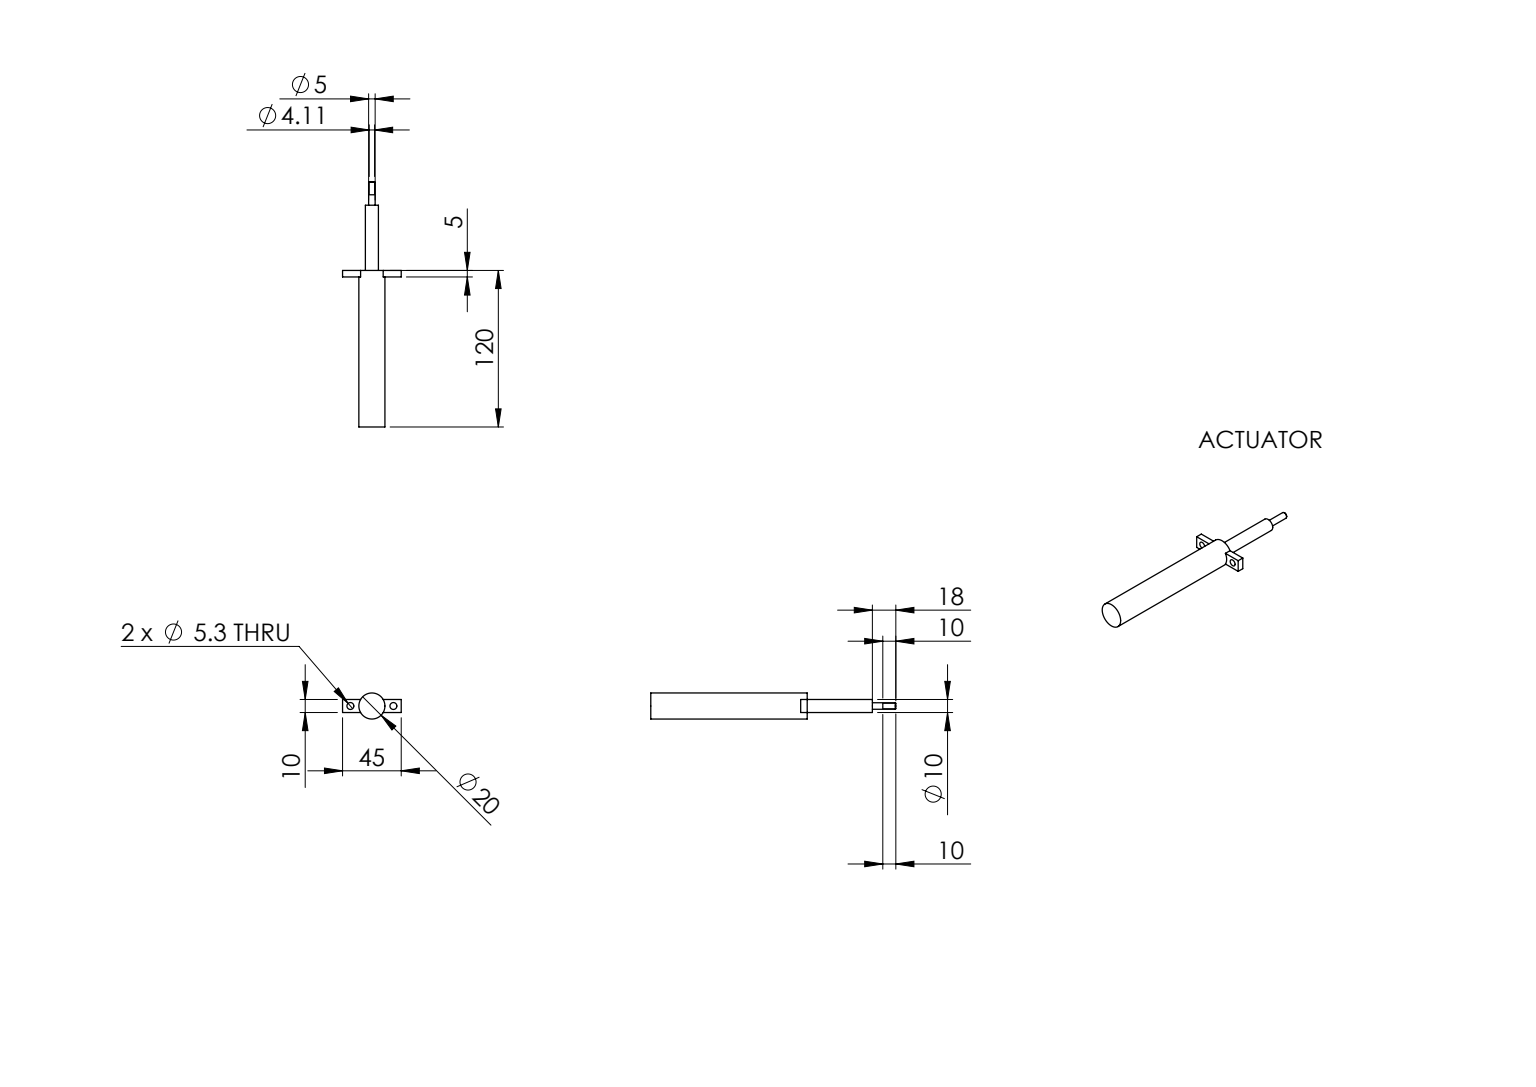
ISO-10303-21;
HEADER;
FILE_DESCRIPTION (('STEP AP214'),
    '1' );
FILE_NAME ('actuator.step',
    '2026-10-24T13:33:06',
    ( '' ),
    ( '' ),
    'SwSTEP 2.0',
    'SolidWorks 2026',
    '' );
FILE_SCHEMA (( 'AUTOMOTIVE_DESIGN' ));
ENDSEC;

DATA;
#20=DIRECTION ( 'NONE',  ( 1.000000000000000000, 0.000000000000000000, 0.000000000000000000 ) ) ;
#34=EDGE_CURVE ( 'NONE', #3584, #3648, #12190, .T. ) ;
#121=ORIENTED_EDGE ( 'NONE', *, *, #4725, .F. ) ;
#127=DIRECTION ( 'NONE',  ( 0.000000000000000000, 0.000000000000000000, 1.000000000000000000 ) ) ;
#157=DIRECTION ( 'NONE',  ( -0.000000000000000000, -0.000000000000000000, 1.000000000000000000 ) ) ;
#162=DIRECTION ( 'NONE',  ( -0.000000000000000000, -0.000000000000000000, 1.000000000000000000 ) ) ;
#163=ADVANCED_FACE ( 'NONE', ( #5247 ), #3288, .T. ) ;
#168=VECTOR ( 'NONE', #12487, 1000.000000000000000 ) ;
#188=EDGE_CURVE ( 'NONE', #1051, #13344, #1074, .T. ) ;
#210=ORIENTED_EDGE ( 'NONE', *, *, #2503, .T. ) ;
#258=VERTEX_POINT ( 'NONE', #13414 ) ;
#274=CARTESIAN_POINT ( 'NONE',  ( 242.5000000000000000, -90.00000000000007105, 55.00000000000001421 ) ) ;
#298=VERTEX_POINT ( 'NONE', #6685 ) ;
#306=EDGE_LOOP ( 'NONE', ( #4499, #12572, #12024, #6931 ) ) ;
#343=ORIENTED_EDGE ( 'NONE', *, *, #8371, .F. ) ;
#394=ADVANCED_FACE ( 'NONE', ( #11247 ), #10594, .F. ) ;
#443=EDGE_CURVE ( 'NONE', #12712, #546, #11238, .T. ) ;
#468=SURFACE_SIDE_STYLE ('',( #3620 ) ) ;
#480=EDGE_LOOP ( 'NONE', ( #9749, #7641, #121, #4547, #3837, #13911, #3499, #11062 ) ) ;
#501=EDGE_LOOP ( 'NONE', ( #3700, #503, #1246, #7982 ) ) ;
#503=ORIENTED_EDGE ( 'NONE', *, *, #10674, .T. ) ;
#509=CIRCLE ( 'NONE', #8650, 9.999999999999980460 ) ;
#531=EDGE_CURVE ( 'NONE', #10688, #3025, #6522, .T. ) ;
#540=CARTESIAN_POINT ( 'NONE',  ( 203.5000000000000000, -85.00000000000007105, 55.00000000000001421 ) ) ;
#546=VERTEX_POINT ( 'NONE', #7599 ) ;
#572=ORIENTED_EDGE ( 'NONE', *, *, #8259, .T. ) ;
#613=EDGE_CURVE ( 'NONE', #4926, #11608, #3124, .T. ) ;
#636=( GEOMETRIC_REPRESENTATION_CONTEXT ( 3 ) GLOBAL_UNCERTAINTY_ASSIGNED_CONTEXT ( ( #7199 ) ) GLOBAL_UNIT_ASSIGNED_CONTEXT ( ( #9242, #8209, #12578 ) ) REPRESENTATION_CONTEXT ( 'NONE', 'WORKASPACE' ) );
#649=VERTEX_POINT ( 'NONE', #8693 ) ;
#674=DIRECTION ( 'NONE',  ( 0.000000000000000000, 0.000000000000000000, -1.000000000000000000 ) ) ;
#682=VERTEX_POINT ( 'NONE', #2166 ) ;
#685=EDGE_CURVE ( 'NONE', #13286, #10688, #9930, .T. ) ;
#743=CARTESIAN_POINT ( 'NONE',  ( 214.9999999999999716, -85.00000000000007105, 64.14213562373096522 ) ) ;
#776=VECTOR ( 'NONE', #9953, 1000.000000000000000 ) ;
#791=VERTEX_POINT ( 'NONE', #4709 ) ;
#799=ADVANCED_FACE ( 'NONE', ( #1417 ), #12246, .F. ) ;
#836=VECTOR ( 'NONE', #2195, 1000.000000000000000 ) ;
#851=ORIENTED_EDGE ( 'NONE', *, *, #1764, .T. ) ;
#856=CARTESIAN_POINT ( 'NONE',  ( 197.5000000000000000, -90.00000000000007105, 55.00000000000001421 ) ) ;
#858=ORIENTED_EDGE ( 'NONE', *, *, #443, .F. ) ;
#859=DIRECTION ( 'NONE',  ( -0.000000000000000000, -0.000000000000000000, -1.000000000000000000 ) ) ;
#867=ORIENTED_EDGE ( 'NONE', *, *, #6061, .T. ) ;
#954=LINE ( 'NONE', #743, #10862 ) ;
#958=CYLINDRICAL_SURFACE ( 'NONE', #7666, 2.649999999999985700 ) ;
#968=EDGE_CURVE ( 'NONE', #546, #10685, #4921, .T. ) ;
#976=ADVANCED_FACE ( 'NONE', ( #12961, #7516, #14185, #4044 ), #6438, .F. ) ;
#978=DIRECTION ( 'NONE',  ( -0.000000000000000000, -0.000000000000000000, 1.000000000000000000 ) ) ;
#996=DIRECTION ( 'NONE',  ( -1.000000000000000000, -2.775557561562893323E-15, 0.000000000000000000 ) ) ;
#1005=DIRECTION ( 'NONE',  ( -0.000000000000000000, -0.000000000000000000, -1.000000000000000000 ) ) ;
#1051=VERTEX_POINT ( 'NONE', #5213 ) ;
#1074=LINE ( 'NONE', #5527, #776 ) ;
#1077=CARTESIAN_POINT ( 'NONE',  ( 229.9999999999999432, -85.00000000000007105, 170.0000000000000000 ) ) ;
#1113=PLANE ( 'NONE',  #4657 ) ;
#1114=FACE_OUTER_BOUND ( 'NONE', #12708, .T. ) ;
#1130=ADVANCED_FACE ( 'NONE', ( #2636, #11413 ), #1113, .F. ) ;
#1180=ORIENTED_EDGE ( 'NONE', *, *, #12121, .F. ) ;
#1212=DIRECTION ( 'NONE',  ( -1.000000000000000000, 0.000000000000000000, 0.000000000000000000 ) ) ;
#1217=DIRECTION ( 'NONE',  ( 2.775557561562893323E-15, -1.000000000000000000, 0.000000000000000000 ) ) ;
#1245=CARTESIAN_POINT ( 'NONE',  ( 233.8499999999999375, -85.00000000000007105, 55.00000000000001421 ) ) ;
#1246=ORIENTED_EDGE ( 'NONE', *, *, #7530, .T. ) ;
#1271=DIRECTION ( 'NONE',  ( 0.000000000000000000, 1.000000000000000000, 0.000000000000000000 ) ) ;
#1280=CARTESIAN_POINT ( 'NONE',  ( 210.0000000000000000, -85.00000000000007105, 55.00000000000002132 ) ) ;
#1282=DIRECTION ( 'NONE',  ( -0.000000000000000000, -0.000000000000000000, 1.000000000000000000 ) ) ;
#1325=CIRCLE ( 'NONE', #11073, 2.649999999999985700 ) ;
#1326=VECTOR ( 'NONE', #5102, 1000.000000000000000 ) ;
#1334=ADVANCED_FACE ( 'NONE', ( #13791, #8424 ), #3863, .F. ) ;
#1403=AXIS2_PLACEMENT_3D ( 'NONE', #4738, #1592, #4667 ) ;
#1410=( GEOMETRIC_REPRESENTATION_CONTEXT ( 3 ) GLOBAL_UNCERTAINTY_ASSIGNED_CONTEXT ( ( #13197 ) ) GLOBAL_UNIT_ASSIGNED_CONTEXT ( ( #9062, #3423, #3835 ) ) REPRESENTATION_CONTEXT ( 'NONE', 'WORKASPACE' ) );
#1411=DIRECTION ( 'NONE',  ( -1.000000000000000000, 0.000000000000000000, 0.000000000000000000 ) ) ;
#1417=FACE_OUTER_BOUND ( 'NONE', #5088, .T. ) ;
#1427=EDGE_CURVE ( 'NONE', #12703, #13122, #7623, .T. ) ;
#1453=DIRECTION ( 'NONE',  ( 1.000000000000000000, 0.000000000000000000, 0.000000000000000000 ) ) ;
#1463=ORIENTED_EDGE ( 'NONE', *, *, #4765, .F. ) ;
#1483=DIRECTION ( 'NONE',  ( 1.000000000000000000, 0.000000000000000000, 0.000000000000000000 ) ) ;
#1486=CARTESIAN_POINT ( 'NONE',  ( 219.9999999999999147, -85.00000000000009948, -17.55500000000000327 ) ) ;
#1489=EDGE_CURVE ( 'NONE', #11495, #5325, #5454, .T. ) ;
#1545=AXIS2_PLACEMENT_3D ( 'NONE', #4006, #10533, #9520 ) ;
#1552=FACE_OUTER_BOUND ( 'NONE', #13347, .T. ) ;
#1562=ORIENTED_EDGE ( 'NONE', *, *, #10674, .F. ) ;
#1580=ORIENTED_EDGE ( 'NONE', *, *, #6064, .T. ) ;
#1592=DIRECTION ( 'NONE',  ( 0.000000000000000000, -1.000000000000000000, 0.000000000000000000 ) ) ;
#1594=CARTESIAN_POINT ( 'NONE',  ( 206.1500000000000057, -85.00000000000007105, 55.00000000000001421 ) ) ;
#1627=FACE_OUTER_BOUND ( 'NONE', #2552, .T. ) ;
#1637=CARTESIAN_POINT ( 'NONE',  ( 222.0549999999999216, -85.00000000000009948, -18.00000000000000355 ) ) ;
#1642=FACE_OUTER_BOUND ( 'NONE', #13415, .T. ) ;
#1654=DIRECTION ( 'NONE',  ( 1.000000000000000000, 0.000000000000000000, 0.000000000000000000 ) ) ;
#1702=ORIENTED_EDGE ( 'NONE', *, *, #4765, .T. ) ;
#1703=CARTESIAN_POINT ( 'NONE',  ( 219.9999999999999716, -85.00000000000007105, 170.0000000000000000 ) ) ;
#1762=AXIS2_PLACEMENT_3D ( 'NONE', #10106, #12144, #3519 ) ;
#1764=EDGE_CURVE ( 'NONE', #649, #298, #8332, .T. ) ;
#1788=EDGE_LOOP ( 'NONE', ( #3445, #8098, #4357, #6788 ) ) ;
#1793=DIRECTION ( 'NONE',  ( 1.000000000000000000, 0.000000000000000000, 0.000000000000000000 ) ) ;
#1802=EDGE_LOOP ( 'NONE', ( #7587, #12705 ) ) ;
#1805=EDGE_LOOP ( 'NONE', ( #3227, #10313 ) ) ;
#1861=AXIS2_PLACEMENT_3D ( 'NONE', #3908, #10435, #11668 ) ;
#1870=PRODUCT_DEFINITION ( 'UNKNOWN', '', #8642, #2767 ) ;
#1881=VERTEX_POINT ( 'NONE', #5371 ) ;
#2003=CIRCLE ( 'NONE', #14082, 2.649999999999985700 ) ;
#2050=CARTESIAN_POINT ( 'NONE',  ( 219.9999999999999147, -85.00000000000009948, -17.55500000000000327 ) ) ;
#2052=CARTESIAN_POINT ( 'NONE',  ( 200.8500000000000227, -85.00000000000007105, 50.00000000000001421 ) ) ;
#2054=EDGE_CURVE ( 'NONE', #13344, #10688, #7295, .T. ) ;
#2062=ORIENTED_EDGE ( 'NONE', *, *, #1427, .F. ) ;
#2152=EDGE_LOOP ( 'NONE', ( #4708, #4758, #4849, #9813, #5810 ) ) ;
#2166=CARTESIAN_POINT ( 'NONE',  ( 228.6602540378443393, -80.00000000000007105, 50.00000000000001421 ) ) ;
#2181=DIRECTION ( 'NONE',  ( -0.000000000000000000, -1.000000000000000000, -0.000000000000000000 ) ) ;
#2183=LINE ( 'NONE', #856, #3860 ) ;
#2195=DIRECTION ( 'NONE',  ( -0.000000000000000000, -0.000000000000000000, 1.000000000000000000 ) ) ;
#2198=DIRECTION ( 'NONE',  ( 0.000000000000000000, 1.000000000000000000, 0.000000000000000000 ) ) ;
#2200=CLOSED_SHELL ( 'NONE', ( #3269, #5695, #3723, #9080, #6131, #163, #11343, #8907, #4814, #1334, #2313, #976, #394, #799, #3827, #1130, #3012, #3741, #6245, #11618, #8182, #11286, #11248, #13792 ) ) ;
#2216=VECTOR ( 'NONE', #10603, 1000.000000000000000 ) ;
#2220=CARTESIAN_POINT ( 'NONE',  ( 228.6602540378443393, -80.00000000000007105, 55.00000000000002132 ) ) ;
#2233=CARTESIAN_POINT ( 'NONE',  ( 197.5000000000000000, -90.00000000000007105, 55.00000000000001421 ) ) ;
#2236=CARTESIAN_POINT ( 'NONE',  ( 219.9999999999999147, -85.00000000000009948, 0.000000000000000000 ) ) ;
#2237=CIRCLE ( 'NONE', #1762, 9.999999999999980460 ) ;
#2250=DIRECTION ( 'NONE',  ( -1.000000000000000000, 0.000000000000000000, 0.000000000000000000 ) ) ;
#2276=VERTEX_POINT ( 'NONE', #5632 ) ;
#2310=EDGE_LOOP ( 'NONE', ( #10390, #4973 ) ) ;
#2313=ADVANCED_FACE ( 'NONE', ( #8604 ), #5418, .T. ) ;
#2343=CARTESIAN_POINT ( 'NONE',  ( 242.5000000000000000, -90.00000000000007105, 55.00000000000001421 ) ) ;
#2374=DIRECTION ( 'NONE',  ( 1.000000000000000000, 0.000000000000000000, 0.000000000000000000 ) ) ;
#2388=CARTESIAN_POINT ( 'NONE',  ( 203.5000000000000000, -85.00000000000007105, 50.00000000000001421 ) ) ;
#2434=DIRECTION ( 'NONE',  ( 1.000000000000000000, 0.000000000000000000, 0.000000000000000000 ) ) ;
#2438=DIRECTION ( 'NONE',  ( -1.000000000000000000, 0.000000000000000000, 0.000000000000000000 ) ) ;
#2442=VECTOR ( 'NONE', #2980, 1000.000000000000000 ) ;
#2448=DIRECTION ( 'NONE',  ( -0.000000000000000000, -0.000000000000000000, 1.000000000000000000 ) ) ;
#2470=AXIS2_PLACEMENT_3D ( 'NONE', #11242, #1282, #9061 ) ;
#2487=VECTOR ( 'NONE', #12138, 1000.000000000000000 ) ;
#2503=EDGE_CURVE ( 'NONE', #3958, #258, #9010, .T. ) ;
#2552=EDGE_LOOP ( 'NONE', ( #4449, #1463, #8826, #1580 ) ) ;
#2566=EDGE_CURVE ( 'NONE', #4150, #298, #9941, .T. ) ;
#2593=DIRECTION ( 'NONE',  ( 1.000000000000000000, 0.000000000000000000, 0.000000000000000000 ) ) ;
#2636=FACE_BOUND ( 'NONE', #1805, .T. ) ;
#2658=EDGE_CURVE ( 'NONE', #3958, #4926, #9300, .T. ) ;
#2668=VECTOR ( 'NONE', #5368, 1000.000000000000000 ) ;
#2690=ORIENTED_EDGE ( 'NONE', *, *, #5877, .T. ) ;
#2693=CARTESIAN_POINT ( 'NONE',  ( 222.0549999999999216, -85.00000000000009948, -18.00000000000000355 ) ) ;
#2714=VECTOR ( 'NONE', #8375, 1000.000000000000000 ) ;
#2741=VERTEX_POINT ( 'NONE', #13500 ) ;
#2767=PRODUCT_DEFINITION_CONTEXT ( 'detailed design', #12304, 'design' ) ;
#2828=CIRCLE ( 'NONE', #10943, 2.500000000000002220 ) ;
#2837=CARTESIAN_POINT ( 'NONE',  ( 242.5000000000000000, -90.00000000000007105, 50.00000000000001421 ) ) ;
#2965=DIRECTION ( 'NONE',  ( 1.000000000000000000, 0.000000000000000000, -0.000000000000000000 ) ) ;
#2980=DIRECTION ( 'NONE',  ( -1.000000000000000000, -0.000000000000000000, -0.000000000000000000 ) ) ;
#3012=ADVANCED_FACE ( 'NONE', ( #4434 ), #8851, .F. ) ;
#3025=VERTEX_POINT ( 'NONE', #14140 ) ;
#3029=DIRECTION ( 'NONE',  ( -1.000000000000000000, 0.000000000000000000, 0.000000000000000000 ) ) ;
#3044=AXIS2_PLACEMENT_3D ( 'NONE', #8830, #12373, #20 ) ;
#3048=CIRCLE ( 'NONE', #13450, 2.055000000000001492 ) ;
#3099=CARTESIAN_POINT ( 'NONE',  ( 219.9999999999999716, -85.00000000000007105, 50.00000000000001421 ) ) ;
#3124=LINE ( 'NONE', #10954, #7740 ) ;
#3168=LINE ( 'NONE', #7360, #2714 ) ;
#3217=VERTEX_POINT ( 'NONE', #1280 ) ;
#3223=ORIENTED_EDGE ( 'NONE', *, *, #11905, .F. ) ;
#3227=ORIENTED_EDGE ( 'NONE', *, *, #8947, .F. ) ;
#3230=FACE_OUTER_BOUND ( 'NONE', #11862, .T. ) ;
#3235=EDGE_CURVE ( 'NONE', #10685, #7175, #9516, .T. ) ;
#3269=ADVANCED_FACE ( 'NONE', ( #1642 ), #11741, .T. ) ;
#3277=DIRECTION ( 'NONE',  ( 0.000000000000000000, 0.000000000000000000, -1.000000000000000000 ) ) ;
#3282=LINE ( 'NONE', #10019, #6027 ) ;
#3288=CYLINDRICAL_SURFACE ( 'NONE', #13312, 9.999999999999980460 ) ;
#3304=FACE_OUTER_BOUND ( 'NONE', #501, .T. ) ;
#3326=VECTOR ( 'NONE', #6308, 1000.000000000000000 ) ;
#3331=CIRCLE ( 'NONE', #8165, 5.000000000000004441 ) ;
#3353=DIRECTION ( 'NONE',  ( 1.000000000000000000, 0.000000000000000000, 0.000000000000000000 ) ) ;
#3362=EDGE_LOOP ( 'NONE', ( #3792, #12684, #11851, #10750 ) ) ;
#3363=DIRECTION ( 'NONE',  ( -1.000000000000000000, 0.000000000000000000, 0.000000000000000000 ) ) ;
#3375=EDGE_LOOP ( 'NONE', ( #9305, #6235 ) ) ;
#3385=SHAPE_REPRESENTATION ( 'actuator', ( #14039 ), #1410 ) ;
#3411=DIRECTION ( 'NONE',  ( 1.000000000000000000, 0.000000000000000000, 0.000000000000000000 ) ) ;
#3423=( NAMED_UNIT ( * ) PLANE_ANGLE_UNIT ( ) SI_UNIT ( $, .RADIAN. ) );
#3439=DIRECTION ( 'NONE',  ( -0.000000000000000000, -0.000000000000000000, 1.000000000000000000 ) ) ;
#3440=DIRECTION ( 'NONE',  ( 1.000000000000000000, 0.000000000000000000, 0.000000000000000000 ) ) ;
#3445=ORIENTED_EDGE ( 'NONE', *, *, #1764, .F. ) ;
#3458=CARTESIAN_POINT ( 'NONE',  ( 242.4999999999999716, -80.00000000000007105, 55.00000000000001421 ) ) ;
#3462=CYLINDRICAL_SURFACE ( 'NONE', #12998, 2.649999999999985700 ) ;
#3466=EDGE_LOOP ( 'NONE', ( #2062, #7298, #14098, #9821, #343, #13771, #1562, #1180 ) ) ;
#3499=ORIENTED_EDGE ( 'NONE', *, *, #4750, .F. ) ;
#3519=DIRECTION ( 'NONE',  ( -1.000000000000000000, 0.000000000000000000, 0.000000000000000000 ) ) ;
#3536=DIRECTION ( 'NONE',  ( -0.000000000000000000, -0.000000000000000000, -1.000000000000000000 ) ) ;
#3561=ORIENTED_EDGE ( 'NONE', *, *, #8052, .T. ) ;
#3584=VERTEX_POINT ( 'NONE', #7278 ) ;
#3602=CYLINDRICAL_SURFACE ( 'NONE', #12776, 2.649999999999985700 ) ;
#3620=SURFACE_STYLE_FILL_AREA ( #12395 ) ;
#3632=ORIENTED_EDGE ( 'NONE', *, *, #11546, .F. ) ;
#3643=CARTESIAN_POINT ( 'NONE',  ( 219.9999999999999716, -85.00000000000007105, 0.000000000000000000 ) ) ;
#3648=VERTEX_POINT ( 'NONE', #2052 ) ;
#3658=EDGE_CURVE ( 'NONE', #649, #13881, #3048, .T. ) ;
#3680=AXIS2_PLACEMENT_3D ( 'NONE', #2050, #8941, #3440 ) ;
#3700=ORIENTED_EDGE ( 'NONE', *, *, #12163, .F. ) ;
#3703=AXIS2_PLACEMENT_3D ( 'NONE', #10869, #10726, #2965 ) ;
#3705=CARTESIAN_POINT ( 'NONE',  ( 239.1499999999999204, -85.00000000000007105, 50.00000000000001421 ) ) ;
#3723=ADVANCED_FACE ( 'NONE', ( #12205 ), #958, .F. ) ;
#3741=ADVANCED_FACE ( 'NONE', ( #3304 ), #10989, .F. ) ;
#3745=CARTESIAN_POINT ( 'NONE',  ( 236.4999999999999432, -85.00000000000007105, 55.00000000000001421 ) ) ;
#3775=DIRECTION ( 'NONE',  ( 1.000000000000000000, 0.000000000000000000, 0.000000000000000000 ) ) ;
#3780=EDGE_LOOP ( 'NONE', ( #12090, #6328, #7485, #8984 ) ) ;
#3787=EDGE_CURVE ( 'NONE', #5325, #2741, #4445, .T. ) ;
#3792=ORIENTED_EDGE ( 'NONE', *, *, #8052, .F. ) ;
#3827=ADVANCED_FACE ( 'NONE', ( #8055 ), #5960, .F. ) ;
#3835=( NAMED_UNIT ( * ) SI_UNIT ( $, .STERADIAN. ) SOLID_ANGLE_UNIT ( ) );
#3837=ORIENTED_EDGE ( 'NONE', *, *, #8504, .T. ) ;
#3860=VECTOR ( 'NONE', #13064, 1000.000000000000000 ) ;
#3863=PLANE ( 'NONE',  #13468 ) ;
#3888=AXIS2_PLACEMENT_3D ( 'NONE', #6533, #14211, #7819 ) ;
#3908=CARTESIAN_POINT ( 'NONE',  ( 236.4999999999999432, -85.00000000000007105, 55.00000000000001421 ) ) ;
#3958=VERTEX_POINT ( 'NONE', #12185 ) ;
#3964=EDGE_CURVE ( 'NONE', #13344, #5408, #3282, .T. ) ;
#3972=PLANE ( 'NONE',  #9753 ) ;
#4006=CARTESIAN_POINT ( 'NONE',  ( 219.9999999999999147, -85.00000000000009948, -17.55500000000000327 ) ) ;
#4035=DIRECTION ( 'NONE',  ( -0.000000000000000000, -0.000000000000000000, -1.000000000000000000 ) ) ;
#4044=FACE_OUTER_BOUND ( 'NONE', #12958, .T. ) ;
#4052=LINE ( 'NONE', #8401, #4402 ) ;
#4083=ORIENTED_EDGE ( 'NONE', *, *, #6289, .T. ) ;
#4099=LINE ( 'NONE', #6128, #11881 ) ;
#4110=CARTESIAN_POINT ( 'NONE',  ( 219.9999999999999716, -85.00000000000007105, 50.00000000000001421 ) ) ;
#4150=VERTEX_POINT ( 'NONE', #8109 ) ;
#4164=DIRECTION ( 'NONE',  ( 1.000000000000000000, 0.000000000000000000, 0.000000000000000000 ) ) ;
#4165=AXIS2_PLACEMENT_3D ( 'NONE', #9623, #674, #14036 ) ;
#4166=DIRECTION ( 'NONE',  ( -0.000000000000000000, -0.000000000000000000, 1.000000000000000000 ) ) ;
#4244=CARTESIAN_POINT ( 'NONE',  ( 210.0000000000000000, -85.00000000000007105, 170.0000000000000000 ) ) ;
#4261=DIRECTION ( 'NONE',  ( 1.000000000000000000, 0.000000000000000000, -0.000000000000000000 ) ) ;
#4287=EDGE_LOOP ( 'NONE', ( #11625, #4346, #13827, #9504 ) ) ;
#4289=DIRECTION ( 'NONE',  ( 0.000000000000000000, -0.000000000000000000, -1.000000000000000000 ) ) ;
#4298=ORIENTED_EDGE ( 'NONE', *, *, #3235, .T. ) ;
#4346=ORIENTED_EDGE ( 'NONE', *, *, #7170, .T. ) ;
#4348=DIRECTION ( 'NONE',  ( -1.000000000000000000, -0.000000000000000000, -0.000000000000000000 ) ) ;
#4357=ORIENTED_EDGE ( 'NONE', *, *, #10565, .T. ) ;
#4386=DIRECTION ( 'NONE',  ( 1.000000000000000000, 0.000000000000000000, 0.000000000000000000 ) ) ;
#4389=CARTESIAN_POINT ( 'NONE',  ( 197.5000000000000000, -90.00000000000007105, 55.00000000000001421 ) ) ;
#4402=VECTOR ( 'NONE', #978, 1000.000000000000000 ) ;
#4434=FACE_OUTER_BOUND ( 'NONE', #3780, .T. ) ;
#4441=ORIENTED_EDGE ( 'NONE', *, *, #11212, .F. ) ;
#4445=CIRCLE ( 'NONE', #8096, 5.000000000000004441 ) ;
#4446=DIRECTION ( 'NONE',  ( -0.000000000000000000, -0.000000000000000000, -1.000000000000000000 ) ) ;
#4449=ORIENTED_EDGE ( 'NONE', *, *, #1489, .F. ) ;
#4469=EDGE_CURVE ( 'NONE', #298, #9222, #4052, .T. ) ;
#4472=ORIENTED_EDGE ( 'NONE', *, *, #11702, .F. ) ;
#4483=DIRECTION ( 'NONE',  ( -1.000000000000000000, 0.000000000000000000, -0.000000000000000000 ) ) ;
#4484=VECTOR ( 'NONE', #10993, 1000.000000000000000 ) ;
#4495=PRODUCT ( 'actuator', 'actuator', '', ( #4956 ) ) ;
#4499=ORIENTED_EDGE ( 'NONE', *, *, #10635, .F. ) ;
#4547=ORIENTED_EDGE ( 'NONE', *, *, #13997, .F. ) ;
#4591=DIRECTION ( 'NONE',  ( -0.000000000000000000, -0.000000000000000000, 1.000000000000000000 ) ) ;
#4595=DIRECTION ( 'NONE',  ( 0.000000000000000000, -0.000000000000000000, 1.000000000000000000 ) ) ;
#4622=CARTESIAN_POINT ( 'NONE',  ( 236.4999999999999432, -85.00000000000007105, 55.00000000000001421 ) ) ;
#4635=ORIENTED_EDGE ( 'NONE', *, *, #6061, .F. ) ;
#4657=AXIS2_PLACEMENT_3D ( 'NONE', #7054, #11084, #4483 ) ;
#4667=DIRECTION ( 'NONE',  ( 0.000000000000000000, -0.000000000000000000, -1.000000000000000000 ) ) ;
#4708=ORIENTED_EDGE ( 'NONE', *, *, #613, .T. ) ;
#4709=CARTESIAN_POINT ( 'NONE',  ( 210.0000000000000000, -85.00000000000007105, 170.0000000000000000 ) ) ;
#4725=EDGE_CURVE ( 'NONE', #11608, #13122, #6473, .T. ) ;
#4738=CARTESIAN_POINT ( 'NONE',  ( 197.5000000000000000, -80.00000000000007105, 55.00000000000001421 ) ) ;
#4750=EDGE_CURVE ( 'NONE', #3217, #1051, #8158, .T. ) ;
#4758=ORIENTED_EDGE ( 'NONE', *, *, #4725, .T. ) ;
#4759=AXIS2_PLACEMENT_3D ( 'NONE', #5349, #7789, #4261 ) ;
#4765=EDGE_CURVE ( 'NONE', #1881, #11495, #7399, .T. ) ;
#4774=DIRECTION ( 'NONE',  ( -0.000000000000000000, -0.000000000000000000, 1.000000000000000000 ) ) ;
#4785=AXIS2_PLACEMENT_3D ( 'NONE', #7078, #10346, #1483 ) ;
#4792=VECTOR ( 'NONE', #8065, 1000.000000000000000 ) ;
#4814=ADVANCED_FACE ( 'NONE', ( #1627 ), #5066, .T. ) ;
#4825=CARTESIAN_POINT ( 'NONE',  ( 200.8500000000000227, -85.00000000000007105, 55.00000000000001421 ) ) ;
#4848=DIRECTION ( 'NONE',  ( -0.000000000000000000, -0.000000000000000000, 1.000000000000000000 ) ) ;
#4849=ORIENTED_EDGE ( 'NONE', *, *, #12121, .T. ) ;
#4853=DIRECTION ( 'NONE',  ( 0.000000000000000000, 0.000000000000000000, -1.000000000000000000 ) ) ;
#4886=ORIENTED_EDGE ( 'NONE', *, *, #2054, .T. ) ;
#4897=LINE ( 'NONE', #9318, #9440 ) ;
#4916=COLOUR_RGB ( '',0.8941176470588234615, 0.8941176470588234615, 0.8941176470588234615 ) ;
#4921=LINE ( 'NONE', #13896, #5342 ) ;
#4926=VERTEX_POINT ( 'NONE', #3458 ) ;
#4956=PRODUCT_CONTEXT ( 'NONE', #6096, 'mechanical' ) ;
#4973=ORIENTED_EDGE ( 'NONE', *, *, #11212, .T. ) ;
#4986=CARTESIAN_POINT ( 'NONE',  ( 219.9999999999999716, -85.00000000000007105, 64.14213562373096522 ) ) ;
#4993=DIRECTION ( 'NONE',  ( -0.000000000000000000, -0.000000000000000000, 1.000000000000000000 ) ) ;
#5013=ORIENTED_EDGE ( 'NONE', *, *, #8715, .F. ) ;
#5019=CIRCLE ( 'NONE', #2470, 2.500000000000002220 ) ;
#5035=AXIS2_PLACEMENT_3D ( 'NONE', #1703, #13676, #11577 ) ;
#5066=CYLINDRICAL_SURFACE ( 'NONE', #8313, 5.000000000000004441 ) ;
#5072=VECTOR ( 'NONE', #11856, 1000.000000000000000 ) ;
#5077=DIRECTION ( 'NONE',  ( 1.000000000000000000, 0.000000000000000000, 0.000000000000000000 ) ) ;
#5088=EDGE_LOOP ( 'NONE', ( #7598, #6594, #6457, #2690 ) ) ;
#5101=EDGE_LOOP ( 'NONE', ( #13141, #5013 ) ) ;
#5102=DIRECTION ( 'NONE',  ( 0.000000000000000000, 0.000000000000000000, 1.000000000000000000 ) ) ;
#5206=ORIENTED_EDGE ( 'NONE', *, *, #34, .T. ) ;
#5213=CARTESIAN_POINT ( 'NONE',  ( 211.3397459621556038, -80.00000000000007105, 55.00000000000002132 ) ) ;
#5245=AXIS2_PLACEMENT_3D ( 'NONE', #2233, #1271, #9118 ) ;
#5247=FACE_OUTER_BOUND ( 'NONE', #480, .T. ) ;
#5258=ADVANCED_BREP_SHAPE_REPRESENTATION ( '', ( #13412, #14039 ), #1410 ) ;
#5264=VECTOR ( 'NONE', #6604, 1000.000000000000000 ) ;
#5309=CARTESIAN_POINT ( 'NONE',  ( 239.1499999999999204, -85.00000000000007105, 55.00000000000001421 ) ) ;
#5325=VERTEX_POINT ( 'NONE', #6124 ) ;
#5342=VECTOR ( 'NONE', #4993, 1000.000000000000000 ) ;
#5349=CARTESIAN_POINT ( 'NONE',  ( 219.9999999999999716, -85.00000000000007105, 170.0000000000000000 ) ) ;
#5368=DIRECTION ( 'NONE',  ( -0.000000000000000000, -1.000000000000000000, -0.000000000000000000 ) ) ;
#5371=CARTESIAN_POINT ( 'NONE',  ( 214.9999999999999716, -85.00000000000007105, 50.00000000000001421 ) ) ;
#5408=VERTEX_POINT ( 'NONE', #4389 ) ;
#5418=PLANE ( 'NONE',  #4759 ) ;
#5454=LINE ( 'NONE', #5599, #10948 ) ;
#5464=LINE ( 'NONE', #4244, #2487 ) ;
#5467=EDGE_CURVE ( 'NONE', #791, #3217, #5464, .T. ) ;
#5468=CARTESIAN_POINT ( 'NONE',  ( 197.5000000000000000, -80.00000000000007105, 50.00000000000001421 ) ) ;
#5512=EDGE_CURVE ( 'NONE', #5681, #13411, #1325, .T. ) ;
#5527=CARTESIAN_POINT ( 'NONE',  ( 197.5000000000000000, -80.00000000000007105, 55.00000000000001421 ) ) ;
#5537=CARTESIAN_POINT ( 'NONE',  ( 219.9999999999999147, -85.00000000000009948, 0.000000000000000000 ) ) ;
#5538=LINE ( 'NONE', #14159, #836 ) ;
#5599=CARTESIAN_POINT ( 'NONE',  ( 224.9999999999999716, -85.00000000000007105, 64.14213562373096522 ) ) ;
#5632=CARTESIAN_POINT ( 'NONE',  ( 211.3397459621556038, -90.00000000000007105, 55.00000000000002132 ) ) ;
#5664=ORIENTED_EDGE ( 'NONE', *, *, #2566, .F. ) ;
#5669=CARTESIAN_POINT ( 'NONE',  ( 203.5000000000000000, -85.00000000000007105, 50.00000000000001421 ) ) ;
#5674=DIRECTION ( 'NONE',  ( -0.000000000000000000, -0.000000000000000000, 1.000000000000000000 ) ) ;
#5681=VERTEX_POINT ( 'NONE', #1594 ) ;
#5695=ADVANCED_FACE ( 'NONE', ( #11690 ), #13137, .T. ) ;
#5701=CARTESIAN_POINT ( 'NONE',  ( 219.9999999999999716, -85.00000000000007105, 170.0000000000000000 ) ) ;
#5722=CARTESIAN_POINT ( 'NONE',  ( 197.5000000000000000, -90.00000000000007105, 55.00000000000001421 ) ) ;
#5737=VERTEX_POINT ( 'NONE', #5964 ) ;
#5748=MECHANICAL_DESIGN_GEOMETRIC_PRESENTATION_REPRESENTATION('',(#10149),#636);
#5796=SHAPE_REPRESENTATION_RELATIONSHIP ( 'NONE' , 'NONE' ,  #3385, #5258 ) ;
#5810=ORIENTED_EDGE ( 'NONE', *, *, #2658, .T. ) ;
#5812=CARTESIAN_POINT ( 'NONE',  ( 222.4999999999999147, -85.00000000000009948, 0.000000000000000000 ) ) ;
#5831=( GEOMETRIC_REPRESENTATION_CONTEXT ( 3 ) GLOBAL_UNCERTAINTY_ASSIGNED_CONTEXT ( ( #7678 ) ) GLOBAL_UNIT_ASSIGNED_CONTEXT ( ( #10513, #11386, #6954 ) ) REPRESENTATION_CONTEXT ( 'NONE', 'WORKASPACE' ) );
#5877=EDGE_CURVE ( 'NONE', #5408, #3025, #2183, .T. ) ;
#5924=DIRECTION ( 'NONE',  ( 0.000000000000000000, 0.000000000000000000, -1.000000000000000000 ) ) ;
#5929=DIRECTION ( 'NONE',  ( 1.000000000000000000, 0.000000000000000000, 0.000000000000000000 ) ) ;
#5960=PLANE ( 'NONE',  #1403 ) ;
#5964=CARTESIAN_POINT ( 'NONE',  ( 211.3397459621556038, -90.00000000000007105, 50.00000000000001421 ) ) ;
#5966=ORIENTED_EDGE ( 'NONE', *, *, #531, .F. ) ;
#5969=AXIS2_PLACEMENT_3D ( 'NONE', #11239, #11107, #3353 ) ;
#5986=EDGE_LOOP ( 'NONE', ( #12619, #12076, #11050, #210 ) ) ;
#6001=FACE_OUTER_BOUND ( 'NONE', #9836, .T. ) ;
#6027=VECTOR ( 'NONE', #2181, 1000.000000000000000 ) ;
#6033=SHAPE_DEFINITION_REPRESENTATION ( #12484, #3385 ) ;
#6036=CONICAL_SURFACE ( 'NONE', #11591, 2.500000000000002220, 0.7853981633974521648 ) ;
#6046=EDGE_LOOP ( 'NONE', ( #5206, #572 ) ) ;
#6059=DIRECTION ( 'NONE',  ( 1.000000000000000000, 0.000000000000000000, 0.000000000000000000 ) ) ;
#6061=EDGE_CURVE ( 'NONE', #13881, #649, #7325, .T. ) ;
#6064=EDGE_CURVE ( 'NONE', #2741, #5325, #8483, .T. ) ;
#6096=APPLICATION_CONTEXT ( 'automotive_design' ) ;
#6124=CARTESIAN_POINT ( 'NONE',  ( 224.9999999999999716, -85.00000000000007105, 0.000000000000000000 ) ) ;
#6128=CARTESIAN_POINT ( 'NONE',  ( 222.4999999999999147, -85.00000000000009948, -17.55500000000000327 ) ) ;
#6131=ADVANCED_FACE ( 'NONE', ( #9480 ), #7228, .T. ) ;
#6132=DIRECTION ( 'NONE',  ( 0.000000000000000000, 0.000000000000000000, 1.000000000000000000 ) ) ;
#6147=PLANE ( 'NONE',  #9041 ) ;
#6182=DIRECTION ( 'NONE',  ( 1.000000000000000000, 0.000000000000000000, -0.000000000000000000 ) ) ;
#6199=EDGE_CURVE ( 'NONE', #5408, #2276, #13407, .T. ) ;
#6235=ORIENTED_EDGE ( 'NONE', *, *, #3787, .F. ) ;
#6241=DIRECTION ( 'NONE',  ( -0.000000000000000000, -0.000000000000000000, -1.000000000000000000 ) ) ;
#6245=ADVANCED_FACE ( 'NONE', ( #8853 ), #10971, .F. ) ;
#6289=EDGE_CURVE ( 'NONE', #298, #4150, #5019, .T. ) ;
#6291=DIRECTION ( 'NONE',  ( 0.000000000000000000, 0.000000000000000000, 1.000000000000000000 ) ) ;
#6308=DIRECTION ( 'NONE',  ( -0.7071067811865502373, 8.659560562354966138E-17, 0.7071067811865447972 ) ) ;
#6328=ORIENTED_EDGE ( 'NONE', *, *, #13997, .T. ) ;
#6329=ORIENTED_EDGE ( 'NONE', *, *, #3964, .F. ) ;
#6361=ORIENTED_EDGE ( 'NONE', *, *, #3964, .T. ) ;
#6365=CARTESIAN_POINT ( 'NONE',  ( 224.9999999999999716, -85.00000000000007105, 50.00000000000001421 ) ) ;
#6407=VECTOR ( 'NONE', #5929, 1000.000000000000000 ) ;
#6431=VECTOR ( 'NONE', #8478, 1000.000000000000000 ) ;
#6438=PLANE ( 'NONE',  #3703 ) ;
#6457=ORIENTED_EDGE ( 'NONE', *, *, #6199, .F. ) ;
#6464=CARTESIAN_POINT ( 'NONE',  ( 197.5000000000000000, -80.00000000000007105, 55.00000000000001421 ) ) ;
#6473=CIRCLE ( 'NONE', #11804, 9.999999999999980460 ) ;
#6500=CARTESIAN_POINT ( 'NONE',  ( 217.4999999999999147, -85.00000000000009948, 0.000000000000000000 ) ) ;
#6501=AXIS2_PLACEMENT_3D ( 'NONE', #8322, #9493, #1793 ) ;
#6522=LINE ( 'NONE', #8623, #2668 ) ;
#6533=CARTESIAN_POINT ( 'NONE',  ( 219.9999999999999716, -85.00000000000007105, 50.00000000000001421 ) ) ;
#6548=CIRCLE ( 'NONE', #8144, 2.649999999999985700 ) ;
#6594=ORIENTED_EDGE ( 'NONE', *, *, #8371, .T. ) ;
#6604=DIRECTION ( 'NONE',  ( 1.000000000000000000, 0.000000000000000000, 0.000000000000000000 ) ) ;
#6649=CARTESIAN_POINT ( 'NONE',  ( 236.4999999999999432, -85.00000000000007105, 55.00000000000001421 ) ) ;
#6685=CARTESIAN_POINT ( 'NONE',  ( 217.4999999999999147, -85.00000000000009948, -17.55500000000000327 ) ) ;
#6704=ORIENTED_EDGE ( 'NONE', *, *, #8018, .F. ) ;
#6738=ORIENTED_EDGE ( 'NONE', *, *, #7024, .T. ) ;
#6776=CARTESIAN_POINT ( 'NONE',  ( 228.6602540378443393, -90.00000000000007105, 170.0000000000000000 ) ) ;
#6788=ORIENTED_EDGE ( 'NONE', *, *, #6289, .F. ) ;
#6823=VERTEX_POINT ( 'NONE', #13221 ) ;
#6835=ORIENTED_EDGE ( 'NONE', *, *, #2566, .T. ) ;
#6931=ORIENTED_EDGE ( 'NONE', *, *, #13208, .F. ) ;
#6933=CARTESIAN_POINT ( 'NONE',  ( 219.9999999999999716, -85.00000000000007105, 55.00000000000002132 ) ) ;
#6947=LINE ( 'NONE', #12538, #6407 ) ;
#6954=( NAMED_UNIT ( * ) SI_UNIT ( $, .STERADIAN. ) SOLID_ANGLE_UNIT ( ) );
#6986=ORIENTED_EDGE ( 'NONE', *, *, #8605, .F. ) ;
#6988=STYLED_ITEM ( 'NONE', ( #9280 ), #5258 ) ;
#7024=EDGE_CURVE ( 'NONE', #4150, #8111, #12409, .T. ) ;
#7050=ORIENTED_EDGE ( 'NONE', *, *, #10635, .T. ) ;
#7054=CARTESIAN_POINT ( 'NONE',  ( 0.000000000000000000, 0.000000000000000000, 55.00000000000001421 ) ) ;
#7070=DIRECTION ( 'NONE',  ( 1.000000000000000000, 0.000000000000000000, 0.000000000000000000 ) ) ;
#7078=CARTESIAN_POINT ( 'NONE',  ( 219.9999999999999716, -85.00000000000007105, 0.000000000000000000 ) ) ;
#7131=ORIENTED_EDGE ( 'NONE', *, *, #9072, .T. ) ;
#7170=EDGE_CURVE ( 'NONE', #1051, #13286, #12556, .T. ) ;
#7175=VERTEX_POINT ( 'NONE', #5309 ) ;
#7199=UNCERTAINTY_MEASURE_WITH_UNIT (LENGTH_MEASURE( 1.000000000000000082E-05 ), #9242, 'distance_accuracy_value', 'NONE');
#7228=CYLINDRICAL_SURFACE ( 'NONE', #8953, 5.000000000000004441 ) ;
#7278=CARTESIAN_POINT ( 'NONE',  ( 206.1500000000000057, -85.00000000000007105, 50.00000000000001421 ) ) ;
#7295=LINE ( 'NONE', #7369, #13660 ) ;
#7298=ORIENTED_EDGE ( 'NONE', *, *, #9072, .F. ) ;
#7325=CIRCLE ( 'NONE', #11974, 2.055000000000001492 ) ;
#7360=CARTESIAN_POINT ( 'NONE',  ( 239.1499999999999204, -85.00000000000007105, 55.00000000000001421 ) ) ;
#7369=CARTESIAN_POINT ( 'NONE',  ( 197.5000000000000000, -80.00000000000007105, 55.00000000000001421 ) ) ;
#7399=CIRCLE ( 'NONE', #11572, 5.000000000000004441 ) ;
#7434=VECTOR ( 'NONE', #6059, 1000.000000000000000 ) ;
#7436=CARTESIAN_POINT ( 'NONE',  ( 197.5000000000000000, -80.00000000000007105, 50.00000000000001421 ) ) ;
#7443=DIRECTION ( 'NONE',  ( -0.000000000000000000, -0.000000000000000000, -1.000000000000000000 ) ) ;
#7477=ORIENTED_EDGE ( 'NONE', *, *, #968, .T. ) ;
#7485=ORIENTED_EDGE ( 'NONE', *, *, #613, .F. ) ;
#7486=CARTESIAN_POINT ( 'NONE',  ( 219.9999999999999716, -85.00000000000007105, 170.0000000000000000 ) ) ;
#7516=FACE_BOUND ( 'NONE', #1802, .T. ) ;
#7530=EDGE_CURVE ( 'NONE', #10602, #258, #6947, .T. ) ;
#7533=ORIENTED_EDGE ( 'NONE', *, *, #4469, .T. ) ;
#7560=VECTOR ( 'NONE', #9471, 1000.000000000000000 ) ;
#7563=DIRECTION ( 'NONE',  ( 1.000000000000000000, 0.000000000000000000, 0.000000000000000000 ) ) ;
#7567=AXIS2_PLACEMENT_3D ( 'NONE', #4622, #162, #2374 ) ;
#7580=AXIS2_PLACEMENT_3D ( 'NONE', #11404, #4591, #11333 ) ;
#7585=AXIS2_PLACEMENT_3D ( 'NONE', #5537, #3439, #12277 ) ;
#7587=ORIENTED_EDGE ( 'NONE', *, *, #443, .T. ) ;
#7598=ORIENTED_EDGE ( 'NONE', *, *, #11702, .T. ) ;
#7599=CARTESIAN_POINT ( 'NONE',  ( 233.8499999999999375, -85.00000000000007105, 50.00000000000001421 ) ) ;
#7623=LINE ( 'NONE', #1077, #11877 ) ;
#7641=ORIENTED_EDGE ( 'NONE', *, *, #1427, .T. ) ;
#7666=AXIS2_PLACEMENT_3D ( 'NONE', #13227, #5674, #4386 ) ;
#7678=UNCERTAINTY_MEASURE_WITH_UNIT (LENGTH_MEASURE( 1.000000000000000082E-05 ), #10513, 'distance_accuracy_value', 'NONE');
#7681=DIRECTION ( 'NONE',  ( 0.000000000000000000, -1.000000000000000000, 0.000000000000000000 ) ) ;
#7701=CARTESIAN_POINT ( 'NONE',  ( 197.5000000000000000, -80.00000000000007105, 50.00000000000001421 ) ) ;
#7740=VECTOR ( 'NONE', #4348, 1000.000000000000000 ) ;
#7789=DIRECTION ( 'NONE',  ( 0.000000000000000000, 0.000000000000000000, 1.000000000000000000 ) ) ;
#7818=CARTESIAN_POINT ( 'NONE',  ( 219.9999999999999716, -85.00000000000007105, 55.00000000000002132 ) ) ;
#7819=DIRECTION ( 'NONE',  ( 1.000000000000000000, 0.000000000000000000, 0.000000000000000000 ) ) ;
#7950=ORIENTED_EDGE ( 'NONE', *, *, #968, .F. ) ;
#7982=ORIENTED_EDGE ( 'NONE', *, *, #2503, .F. ) ;
#8018=EDGE_CURVE ( 'NONE', #3584, #5681, #4897, .T. ) ;
#8052=EDGE_CURVE ( 'NONE', #3648, #13411, #5538, .T. ) ;
#8055=FACE_OUTER_BOUND ( 'NONE', #4287, .T. ) ;
#8065=DIRECTION ( 'NONE',  ( 1.000000000000000000, 0.000000000000000000, 0.000000000000000000 ) ) ;
#8096=AXIS2_PLACEMENT_3D ( 'NONE', #3643, #9373, #9226 ) ;
#8098=ORIENTED_EDGE ( 'NONE', *, *, #3658, .T. ) ;
#8106=SURFACE_STYLE_USAGE ( .BOTH. , #468 ) ;
#8109=CARTESIAN_POINT ( 'NONE',  ( 222.4999999999999147, -85.00000000000009948, -17.55500000000000327 ) ) ;
#8111=VERTEX_POINT ( 'NONE', #13223 ) ;
#8144=AXIS2_PLACEMENT_3D ( 'NONE', #8221, #6132, #7070 ) ;
#8158=CIRCLE ( 'NONE', #4165, 9.999999999999980460 ) ;
#8165=AXIS2_PLACEMENT_3D ( 'NONE', #3099, #14099, #10854 ) ;
#8182=ADVANCED_FACE ( 'NONE', ( #11858 ), #13012, .F. ) ;
#8209=( NAMED_UNIT ( * ) PLANE_ANGLE_UNIT ( ) SI_UNIT ( $, .RADIAN. ) );
#8221=CARTESIAN_POINT ( 'NONE',  ( 236.4999999999999432, -85.00000000000007105, 50.00000000000001421 ) ) ;
#8259=EDGE_CURVE ( 'NONE', #3648, #3584, #11991, .T. ) ;
#8303=ORIENTED_EDGE ( 'NONE', *, *, #11930, .F. ) ;
#8313=AXIS2_PLACEMENT_3D ( 'NONE', #4986, #7443, #3029 ) ;
#8322=CARTESIAN_POINT ( 'NONE',  ( 219.9999999999999147, -85.00000000000009948, 0.000000000000000000 ) ) ;
#8327=ORIENTED_EDGE ( 'NONE', *, *, #8715, .T. ) ;
#8332=LINE ( 'NONE', #9506, #3326 ) ;
#8371=EDGE_CURVE ( 'NONE', #5737, #2276, #11614, .T. ) ;
#8375=DIRECTION ( 'NONE',  ( -0.000000000000000000, -0.000000000000000000, 1.000000000000000000 ) ) ;
#8388=CARTESIAN_POINT ( 'NONE',  ( 0.000000000000000000, 0.000000000000000000, 55.00000000000001421 ) ) ;
#8401=CARTESIAN_POINT ( 'NONE',  ( 217.4999999999999147, -85.00000000000009948, 0.000000000000000000 ) ) ;
#8403=CARTESIAN_POINT ( 'NONE',  ( 236.4999999999999432, -85.00000000000007105, 50.00000000000001421 ) ) ;
#8405=DIRECTION ( 'NONE',  ( 0.000000000000000000, 0.000000000000000000, 1.000000000000000000 ) ) ;
#8424=FACE_OUTER_BOUND ( 'NONE', #3375, .T. ) ;
#8471=DIRECTION ( 'NONE',  ( 0.000000000000000000, 0.000000000000000000, -1.000000000000000000 ) ) ;
#8478=DIRECTION ( 'NONE',  ( -2.775557561562892929E-15, 1.000000000000000000, 0.000000000000000000 ) ) ;
#8483=CIRCLE ( 'NONE', #4785, 5.000000000000004441 ) ;
#8504=EDGE_CURVE ( 'NONE', #682, #13286, #13155, .T. ) ;
#8604=FACE_OUTER_BOUND ( 'NONE', #9819, .T. ) ;
#8605=EDGE_CURVE ( 'NONE', #5737, #10602, #11303, .T. ) ;
#8623=CARTESIAN_POINT ( 'NONE',  ( 197.5000000000000000, -90.00000000000007105, 50.00000000000001421 ) ) ;
#8633=CARTESIAN_POINT ( 'NONE',  ( 211.3397459621556038, -80.00000000000007105, 170.0000000000000000 ) ) ;
#8642=PRODUCT_DEFINITION_FORMATION_WITH_SPECIFIED_SOURCE ( 'ANY', '', #4495, .NOT_KNOWN. ) ;
#8650=AXIS2_PLACEMENT_3D ( 'NONE', #10597, #8405, #1654 ) ;
#8693=CARTESIAN_POINT ( 'NONE',  ( 217.9449999999999079, -85.00000000000009948, -18.00000000000000355 ) ) ;
#8715=EDGE_CURVE ( 'NONE', #13411, #5681, #2003, .T. ) ;
#8726=VECTOR ( 'NONE', #6241, 1000.000000000000000 ) ;
#8751=AXIS2_PLACEMENT_3D ( 'NONE', #7818, #3277, #1212 ) ;
#8826=ORIENTED_EDGE ( 'NONE', *, *, #13208, .T. ) ;
#8830=CARTESIAN_POINT ( 'NONE',  ( 219.9999999999999147, -85.00000000000009948, 0.000000000000000000 ) ) ;
#8834=CARTESIAN_POINT ( 'NONE',  ( 228.6602540378443393, -90.00000000000007105, 55.00000000000002132 ) ) ;
#8844=MECHANICAL_DESIGN_GEOMETRIC_PRESENTATION_REPRESENTATION('',(#6988),#5831);
#8851=PLANE ( 'NONE',  #13542 ) ;
#8853=FACE_OUTER_BOUND ( 'NONE', #5986, .T. ) ;
#8907=ADVANCED_FACE ( 'NONE', ( #12311 ), #11298, .T. ) ;
#8921=VECTOR ( 'NONE', #10912, 1000.000000000000000 ) ;
#8925=CARTESIAN_POINT ( 'NONE',  ( 219.9999999999999716, -85.00000000000007105, 64.14213562373096522 ) ) ;
#8941=DIRECTION ( 'NONE',  ( -0.000000000000000000, -0.000000000000000000, 1.000000000000000000 ) ) ;
#8947=EDGE_CURVE ( 'NONE', #7175, #10685, #11504, .T. ) ;
#8953=AXIS2_PLACEMENT_3D ( 'NONE', #8925, #11037, #2250 ) ;
#8984=ORIENTED_EDGE ( 'NONE', *, *, #13560, .T. ) ;
#9002=VERTEX_POINT ( 'NONE', #8834 ) ;
#9010=LINE ( 'NONE', #2343, #8921 ) ;
#9041=AXIS2_PLACEMENT_3D ( 'NONE', #1637, #4853, #13684 ) ;
#9061=DIRECTION ( 'NONE',  ( 1.000000000000000000, 0.000000000000000000, 0.000000000000000000 ) ) ;
#9062=( LENGTH_UNIT ( ) NAMED_UNIT ( * ) SI_UNIT ( .MILLI., .METRE. ) );
#9072=EDGE_CURVE ( 'NONE', #791, #12703, #11279, .T. ) ;
#9076=LINE ( 'NONE', #12915, #9903 ) ;
#9080=ADVANCED_FACE ( 'NONE', ( #1552 ), #3602, .F. ) ;
#9118=DIRECTION ( 'NONE',  ( 0.000000000000000000, -0.000000000000000000, 1.000000000000000000 ) ) ;
#9222=VERTEX_POINT ( 'NONE', #6500 ) ;
#9226=DIRECTION ( 'NONE',  ( 1.000000000000000000, 0.000000000000000000, 0.000000000000000000 ) ) ;
#9242=( LENGTH_UNIT ( ) NAMED_UNIT ( * ) SI_UNIT ( .MILLI., .METRE. ) );
#9270=FACE_OUTER_BOUND ( 'NONE', #1788, .T. ) ;
#9280=PRESENTATION_STYLE_ASSIGNMENT (( #8106 ) ) ;
#9300=LINE ( 'NONE', #274, #168 ) ;
#9305=ORIENTED_EDGE ( 'NONE', *, *, #6064, .F. ) ;
#9318=CARTESIAN_POINT ( 'NONE',  ( 206.1500000000000057, -85.00000000000007105, 55.00000000000001421 ) ) ;
#9373=DIRECTION ( 'NONE',  ( 0.000000000000000000, 0.000000000000000000, 1.000000000000000000 ) ) ;
#9418=DIRECTION ( 'NONE',  ( 0.000000000000000000, 0.000000000000000000, 1.000000000000000000 ) ) ;
#9423=FILL_AREA_STYLE_COLOUR ( '', #4916 ) ;
#9440=VECTOR ( 'NONE', #12641, 1000.000000000000000 ) ;
#9469=CARTESIAN_POINT ( 'NONE',  ( 228.6602540378443393, -90.00000000000007105, 50.00000000000001421 ) ) ;
#9471=DIRECTION ( 'NONE',  ( -1.000000000000000000, -0.000000000000000000, -0.000000000000000000 ) ) ;
#9480=FACE_OUTER_BOUND ( 'NONE', #306, .T. ) ;
#9493=DIRECTION ( 'NONE',  ( -0.000000000000000000, -0.000000000000000000, 1.000000000000000000 ) ) ;
#9504=ORIENTED_EDGE ( 'NONE', *, *, #2054, .F. ) ;
#9506=CARTESIAN_POINT ( 'NONE',  ( 217.4999999999999147, -85.00000000000009948, -17.55500000000000327 ) ) ;
#9509=LINE ( 'NONE', #2837, #6431 ) ;
#9516=CIRCLE ( 'NONE', #1861, 2.649999999999985700 ) ;
#9520=DIRECTION ( 'NONE',  ( 1.000000000000000000, 0.000000000000000000, 0.000000000000000000 ) ) ;
#9570=DIRECTION ( 'NONE',  ( 1.000000000000000000, 0.000000000000000000, 0.000000000000000000 ) ) ;
#9585=EDGE_LOOP ( 'NONE', ( #867, #851, #5664, #12091 ) ) ;
#9623=CARTESIAN_POINT ( 'NONE',  ( 219.9999999999999716, -85.00000000000007105, 55.00000000000002132 ) ) ;
#9670=ORIENTED_EDGE ( 'NONE', *, *, #12800, .F. ) ;
#9749=ORIENTED_EDGE ( 'NONE', *, *, #10861, .F. ) ;
#9753=AXIS2_PLACEMENT_3D ( 'NONE', #8388, #5924, #13824 ) ;
#9813=ORIENTED_EDGE ( 'NONE', *, *, #12163, .T. ) ;
#9817=ORIENTED_EDGE ( 'NONE', *, *, #6199, .T. ) ;
#9819=EDGE_LOOP ( 'NONE', ( #7131, #11003 ) ) ;
#9821=ORIENTED_EDGE ( 'NONE', *, *, #14193, .F. ) ;
#9836=EDGE_LOOP ( 'NONE', ( #4635, #10901 ) ) ;
#9903=VECTOR ( 'NONE', #13993, 1000.000000000000000 ) ;
#9930=LINE ( 'NONE', #7701, #2442 ) ;
#9941=CIRCLE ( 'NONE', #3680, 2.500000000000002220 ) ;
#9953=DIRECTION ( 'NONE',  ( -1.000000000000000000, -0.000000000000000000, -0.000000000000000000 ) ) ;
#9975=AXIS2_PLACEMENT_3D ( 'NONE', #13357, #2198, #4595 ) ;
#10019=CARTESIAN_POINT ( 'NONE',  ( 197.5000000000000000, -90.00000000000007105, 55.00000000000001421 ) ) ;
#10106=CARTESIAN_POINT ( 'NONE',  ( 219.9999999999999716, -85.00000000000007105, 55.00000000000002132 ) ) ;
#10111=CARTESIAN_POINT ( 'NONE',  ( 211.3397459621556038, -80.00000000000007105, 50.00000000000001421 ) ) ;
#10149=STYLED_ITEM('',(#14424),#13412);
#10245=ORIENTED_EDGE ( 'NONE', *, *, #8259, .F. ) ;
#10302=EDGE_CURVE ( 'NONE', #546, #12712, #6548, .T. ) ;
#10310=AXIS2_PLACEMENT_3D ( 'NONE', #10517, #13698, #8471 ) ;
#10313=ORIENTED_EDGE ( 'NONE', *, *, #3235, .F. ) ;
#10332=CIRCLE ( 'NONE', #8751, 9.999999999999980460 ) ;
#10335=CARTESIAN_POINT ( 'NONE',  ( 229.9999999999999432, -85.00000000000007105, 55.00000000000002132 ) ) ;
#10346=DIRECTION ( 'NONE',  ( 0.000000000000000000, 0.000000000000000000, 1.000000000000000000 ) ) ;
#10390=ORIENTED_EDGE ( 'NONE', *, *, #11546, .T. ) ;
#10435=DIRECTION ( 'NONE',  ( -0.000000000000000000, -0.000000000000000000, 1.000000000000000000 ) ) ;
#10490=LINE ( 'NONE', #10560, #7434 ) ;
#10505=FACE_BOUND ( 'NONE', #5101, .T. ) ;
#10508=CARTESIAN_POINT ( 'NONE',  ( 0.000000000000000000, 0.000000000000000000, 0.000000000000000000 ) ) ;
#10513=( LENGTH_UNIT ( ) NAMED_UNIT ( * ) SI_UNIT ( .MILLI., .METRE. ) );
#10517=CARTESIAN_POINT ( 'NONE',  ( 197.5000000000000000, -90.00000000000007105, 55.00000000000001421 ) ) ;
#10533=DIRECTION ( 'NONE',  ( -0.000000000000000000, -0.000000000000000000, 1.000000000000000000 ) ) ;
#10560=CARTESIAN_POINT ( 'NONE',  ( 197.5000000000000000, -90.00000000000007105, 50.00000000000001421 ) ) ;
#10565=EDGE_CURVE ( 'NONE', #13881, #4150, #4099, .T. ) ;
#10594=PLANE ( 'NONE',  #10310 ) ;
#10597=CARTESIAN_POINT ( 'NONE',  ( 219.9999999999999716, -85.00000000000007105, 170.0000000000000000 ) ) ;
#10602=VERTEX_POINT ( 'NONE', #9469 ) ;
#10603=DIRECTION ( 'NONE',  ( -0.000000000000000000, -0.000000000000000000, 1.000000000000000000 ) ) ;
#10635=EDGE_CURVE ( 'NONE', #11495, #1881, #3331, .T. ) ;
#10674=EDGE_CURVE ( 'NONE', #9002, #10602, #12011, .T. ) ;
#10685=VERTEX_POINT ( 'NONE', #1245 ) ;
#10687=EDGE_LOOP ( 'NONE', ( #1702, #7050 ) ) ;
#10688=VERTEX_POINT ( 'NONE', #5468 ) ;
#10691=DIRECTION ( 'NONE',  ( 0.000000000000000000, 0.000000000000000000, 1.000000000000000000 ) ) ;
#10726=DIRECTION ( 'NONE',  ( 0.000000000000000000, 0.000000000000000000, 1.000000000000000000 ) ) ;
#10750=ORIENTED_EDGE ( 'NONE', *, *, #5512, .T. ) ;
#10834=EDGE_LOOP ( 'NONE', ( #9817, #13507, #11652, #11928, #6361 ) ) ;
#10854=DIRECTION ( 'NONE',  ( 1.000000000000000000, 0.000000000000000000, 0.000000000000000000 ) ) ;
#10861=EDGE_CURVE ( 'NONE', #12703, #791, #509, .T. ) ;
#10862=VECTOR ( 'NONE', #4035, 1000.000000000000000 ) ;
#10869=CARTESIAN_POINT ( 'NONE',  ( 219.9999999999999716, -85.00000000000007105, 50.00000000000001421 ) ) ;
#10901=ORIENTED_EDGE ( 'NONE', *, *, #3658, .F. ) ;
#10912=DIRECTION ( 'NONE',  ( -0.000000000000000000, -0.000000000000000000, -1.000000000000000000 ) ) ;
#10943=AXIS2_PLACEMENT_3D ( 'NONE', #2236, #2448, #3411 ) ;
#10948=VECTOR ( 'NONE', #1005, 1000.000000000000000 ) ;
#10954=CARTESIAN_POINT ( 'NONE',  ( 197.5000000000000000, -80.00000000000007105, 55.00000000000001421 ) ) ;
#10971=PLANE ( 'NONE',  #11267 ) ;
#10989=PLANE ( 'NONE',  #9975 ) ;
#10993=DIRECTION ( 'NONE',  ( -0.000000000000000000, -0.000000000000000000, -1.000000000000000000 ) ) ;
#11003=ORIENTED_EDGE ( 'NONE', *, *, #10861, .T. ) ;
#11019=ORIENTED_EDGE ( 'NONE', *, *, #531, .T. ) ;
#11037=DIRECTION ( 'NONE',  ( -0.000000000000000000, -0.000000000000000000, -1.000000000000000000 ) ) ;
#11050=ORIENTED_EDGE ( 'NONE', *, *, #2658, .F. ) ;
#11062=ORIENTED_EDGE ( 'NONE', *, *, #5467, .F. ) ;
#11063=EDGE_LOOP ( 'NONE', ( #10245, #3561, #8327, #6704 ) ) ;
#11073=AXIS2_PLACEMENT_3D ( 'NONE', #14096, #4166, #7563 ) ;
#11084=DIRECTION ( 'NONE',  ( 0.000000000000000000, 0.000000000000000000, -1.000000000000000000 ) ) ;
#11107=DIRECTION ( 'NONE',  ( 0.000000000000000000, 0.000000000000000000, 1.000000000000000000 ) ) ;
#11132=ORIENTED_EDGE ( 'NONE', *, *, #4469, .F. ) ;
#11173=CARTESIAN_POINT ( 'NONE',  ( 242.5000000000000000, -90.00000000000007105, 55.00000000000001421 ) ) ;
#11186=ORIENTED_EDGE ( 'NONE', *, *, #11905, .T. ) ;
#11211=CARTESIAN_POINT ( 'NONE',  ( 197.5000000000000000, -80.00000000000007105, 55.00000000000001421 ) ) ;
#11212=EDGE_CURVE ( 'NONE', #9222, #8111, #2828, .T. ) ;
#11238=CIRCLE ( 'NONE', #14014, 2.649999999999985700 ) ;
#11239=CARTESIAN_POINT ( 'NONE',  ( 219.9999999999999716, -85.00000000000007105, 50.00000000000001421 ) ) ;
#11242=CARTESIAN_POINT ( 'NONE',  ( 219.9999999999999147, -85.00000000000009948, -17.55500000000000327 ) ) ;
#11247=FACE_OUTER_BOUND ( 'NONE', #12302, .T. ) ;
#11248=ADVANCED_FACE ( 'NONE', ( #9270 ), #6036, .T. ) ;
#11256=CYLINDRICAL_SURFACE ( 'NONE', #7585, 2.500000000000002220 ) ;
#11267=AXIS2_PLACEMENT_3D ( 'NONE', #11173, #996, #1217 ) ;
#11279=CIRCLE ( 'NONE', #5035, 9.999999999999980460 ) ;
#11286=ADVANCED_FACE ( 'NONE', ( #6001 ), #6147, .T. ) ;
#11298=CYLINDRICAL_SURFACE ( 'NONE', #12230, 9.999999999999980460 ) ;
#11300=DIRECTION ( 'NONE',  ( 0.000000000000000000, 0.000000000000000000, -1.000000000000000000 ) ) ;
#11303=CIRCLE ( 'NONE', #5969, 9.999999999999980460 ) ;
#11307=ORIENTED_EDGE ( 'NONE', *, *, #8947, .T. ) ;
#11333=DIRECTION ( 'NONE',  ( 1.000000000000000000, 0.000000000000000000, 0.000000000000000000 ) ) ;
#11343=ADVANCED_FACE ( 'NONE', ( #11374, #10505 ), #3972, .F. ) ;
#11374=FACE_OUTER_BOUND ( 'NONE', #10834, .T. ) ;
#11386=( NAMED_UNIT ( * ) PLANE_ANGLE_UNIT ( ) SI_UNIT ( $, .RADIAN. ) );
#11404=CARTESIAN_POINT ( 'NONE',  ( 203.5000000000000000, -85.00000000000007105, 55.00000000000001421 ) ) ;
#11413=FACE_OUTER_BOUND ( 'NONE', #2152, .T. ) ;
#11465=ORIENTED_EDGE ( 'NONE', *, *, #7530, .F. ) ;
#11479=ORIENTED_EDGE ( 'NONE', *, *, #8504, .F. ) ;
#11495=VERTEX_POINT ( 'NONE', #6365 ) ;
#11504=CIRCLE ( 'NONE', #7567, 2.649999999999985700 ) ;
#11514=DIRECTION ( 'NONE',  ( 1.000000000000000000, 0.000000000000000000, 0.000000000000000000 ) ) ;
#11546=EDGE_CURVE ( 'NONE', #8111, #9222, #13235, .T. ) ;
#11572=AXIS2_PLACEMENT_3D ( 'NONE', #4110, #13969, #12737 ) ;
#11577=DIRECTION ( 'NONE',  ( 1.000000000000000000, 0.000000000000000000, 0.000000000000000000 ) ) ;
#11591=AXIS2_PLACEMENT_3D ( 'NONE', #1486, #4774, #11514 ) ;
#11608=VERTEX_POINT ( 'NONE', #2220 ) ;
#11614=LINE ( 'NONE', #13782, #1326 ) ;
#11618=ADVANCED_FACE ( 'NONE', ( #1114 ), #3462, .F. ) ;
#11625=ORIENTED_EDGE ( 'NONE', *, *, #188, .F. ) ;
#11652=ORIENTED_EDGE ( 'NONE', *, *, #4750, .T. ) ;
#11668=DIRECTION ( 'NONE',  ( 1.000000000000000000, 0.000000000000000000, 0.000000000000000000 ) ) ;
#11690=FACE_OUTER_BOUND ( 'NONE', #9585, .T. ) ;
#11702=EDGE_CURVE ( 'NONE', #3025, #5737, #10490, .T. ) ;
#11741=CYLINDRICAL_SURFACE ( 'NONE', #6501, 2.500000000000002220 ) ;
#11774=CARTESIAN_POINT ( 'NONE',  ( 219.9999999999999716, -85.00000000000007105, 0.000000000000000000 ) ) ;
#11800=DIRECTION ( 'NONE',  ( -0.000000000000000000, -0.000000000000000000, -1.000000000000000000 ) ) ;
#11804=AXIS2_PLACEMENT_3D ( 'NONE', #6933, #11300, #1411 ) ;
#11851=ORIENTED_EDGE ( 'NONE', *, *, #8018, .T. ) ;
#11856=DIRECTION ( 'NONE',  ( -0.000000000000000000, -0.000000000000000000, -1.000000000000000000 ) ) ;
#11858=FACE_OUTER_BOUND ( 'NONE', #3362, .T. ) ;
#11862=EDGE_LOOP ( 'NONE', ( #11132, #4083, #6738, #4441 ) ) ;
#11867=LINE ( 'NONE', #7436, #7560 ) ;
#11877=VECTOR ( 'NONE', #4446, 1000.000000000000000 ) ;
#11881=VECTOR ( 'NONE', #12945, 1000.000000000000000 ) ;
#11905=EDGE_CURVE ( 'NONE', #12712, #7175, #3168, .T. ) ;
#11908=ORIENTED_EDGE ( 'NONE', *, *, #7024, .F. ) ;
#11928=ORIENTED_EDGE ( 'NONE', *, *, #188, .T. ) ;
#11930=EDGE_CURVE ( 'NONE', #6823, #682, #11867, .T. ) ;
#11974=AXIS2_PLACEMENT_3D ( 'NONE', #12526, #4848, #2593 ) ;
#11991=CIRCLE ( 'NONE', #13587, 2.649999999999985700 ) ;
#12011=LINE ( 'NONE', #6776, #4484 ) ;
#12024=ORIENTED_EDGE ( 'NONE', *, *, #3787, .T. ) ;
#12076=ORIENTED_EDGE ( 'NONE', *, *, #13560, .F. ) ;
#12080=ORIENTED_EDGE ( 'NONE', *, *, #10302, .F. ) ;
#12090=ORIENTED_EDGE ( 'NONE', *, *, #11930, .T. ) ;
#12091=ORIENTED_EDGE ( 'NONE', *, *, #10565, .F. ) ;
#12121=EDGE_CURVE ( 'NONE', #13122, #9002, #2237, .T. ) ;
#12138=DIRECTION ( 'NONE',  ( -0.000000000000000000, -0.000000000000000000, -1.000000000000000000 ) ) ;
#12144=DIRECTION ( 'NONE',  ( 0.000000000000000000, 0.000000000000000000, -1.000000000000000000 ) ) ;
#12163=EDGE_CURVE ( 'NONE', #9002, #3958, #12636, .T. ) ;
#12185=CARTESIAN_POINT ( 'NONE',  ( 242.5000000000000000, -90.00000000000007105, 55.00000000000001421 ) ) ;
#12190=CIRCLE ( 'NONE', #12882, 2.649999999999985700 ) ;
#12205=FACE_OUTER_BOUND ( 'NONE', #11063, .T. ) ;
#12230=AXIS2_PLACEMENT_3D ( 'NONE', #5701, #3536, #2438 ) ;
#12246=PLANE ( 'NONE',  #5245 ) ;
#12277=DIRECTION ( 'NONE',  ( 1.000000000000000000, 0.000000000000000000, 0.000000000000000000 ) ) ;
#12302=EDGE_LOOP ( 'NONE', ( #11019, #13432, #6329, #4886 ) ) ;
#12304=APPLICATION_CONTEXT ( 'automotive_design' ) ;
#12311=FACE_OUTER_BOUND ( 'NONE', #3466, .T. ) ;
#12373=DIRECTION ( 'NONE',  ( -0.000000000000000000, -0.000000000000000000, 1.000000000000000000 ) ) ;
#12395=FILL_AREA_STYLE ('',( #9423 ) ) ;
#12409=LINE ( 'NONE', #5812, #2216 ) ;
#12484=PRODUCT_DEFINITION_SHAPE ( 'NONE', 'NONE',  #1870 ) ;
#12487=DIRECTION ( 'NONE',  ( -2.775557561562892929E-15, 1.000000000000000000, 0.000000000000000000 ) ) ;
#12526=CARTESIAN_POINT ( 'NONE',  ( 219.9999999999999147, -85.00000000000009948, -18.00000000000000355 ) ) ;
#12538=CARTESIAN_POINT ( 'NONE',  ( 197.5000000000000000, -90.00000000000007105, 50.00000000000001421 ) ) ;
#12540=DIRECTION ( 'NONE',  ( 1.000000000000000000, 0.000000000000000000, 0.000000000000000000 ) ) ;
#12556=LINE ( 'NONE', #8633, #8726 ) ;
#12572=ORIENTED_EDGE ( 'NONE', *, *, #1489, .T. ) ;
#12578=( NAMED_UNIT ( * ) SI_UNIT ( $, .STERADIAN. ) SOLID_ANGLE_UNIT ( ) );
#12613=DIRECTION ( 'NONE',  ( 0.000000000000000000, 0.000000000000000000, 1.000000000000000000 ) ) ;
#12619=ORIENTED_EDGE ( 'NONE', *, *, #12800, .T. ) ;
#12636=LINE ( 'NONE', #12713, #4792 ) ;
#12641=DIRECTION ( 'NONE',  ( -0.000000000000000000, -0.000000000000000000, 1.000000000000000000 ) ) ;
#12658=DIRECTION ( 'NONE',  ( 1.000000000000000000, 0.000000000000000000, 0.000000000000000000 ) ) ;
#12684=ORIENTED_EDGE ( 'NONE', *, *, #34, .F. ) ;
#12703=VERTEX_POINT ( 'NONE', #13629 ) ;
#12705=ORIENTED_EDGE ( 'NONE', *, *, #10302, .T. ) ;
#12708=EDGE_LOOP ( 'NONE', ( #7950, #858, #11186, #11307 ) ) ;
#12712=VERTEX_POINT ( 'NONE', #3705 ) ;
#12713=CARTESIAN_POINT ( 'NONE',  ( 197.5000000000000000, -90.00000000000007105, 55.00000000000001421 ) ) ;
#12735=DIRECTION ( 'NONE',  ( -0.000000000000000000, -0.000000000000000000, 1.000000000000000000 ) ) ;
#12737=DIRECTION ( 'NONE',  ( 1.000000000000000000, 0.000000000000000000, 0.000000000000000000 ) ) ;
#12776=AXIS2_PLACEMENT_3D ( 'NONE', #3745, #12735, #12658 ) ;
#12800=EDGE_CURVE ( 'NONE', #258, #6823, #9509, .T. ) ;
#12857=CARTESIAN_POINT ( 'NONE',  ( 242.4999999999999716, -80.00000000000007105, 55.00000000000001421 ) ) ;
#12882=AXIS2_PLACEMENT_3D ( 'NONE', #2388, #6291, #9570 ) ;
#12915=CARTESIAN_POINT ( 'NONE',  ( 228.6602540378443393, -80.00000000000007105, 170.0000000000000000 ) ) ;
#12945=DIRECTION ( 'NONE',  ( 0.7071067811865502373, 0.000000000000000000, 0.7071067811865447972 ) ) ;
#12958=EDGE_LOOP ( 'NONE', ( #11479, #8303, #9670, #11465, #6986, #4472, #5966, #13168 ) ) ;
#12961=FACE_BOUND ( 'NONE', #6046, .T. ) ;
#12998=AXIS2_PLACEMENT_3D ( 'NONE', #6649, #157, #2434 ) ;
#13012=CYLINDRICAL_SURFACE ( 'NONE', #7580, 2.649999999999985700 ) ;
#13064=DIRECTION ( 'NONE',  ( -0.000000000000000000, -0.000000000000000000, -1.000000000000000000 ) ) ;
#13122=VERTEX_POINT ( 'NONE', #10335 ) ;
#13137=CONICAL_SURFACE ( 'NONE', #1545, 2.500000000000002220, 0.7853981633974521648 ) ;
#13141=ORIENTED_EDGE ( 'NONE', *, *, #5512, .F. ) ;
#13155=CIRCLE ( 'NONE', #3888, 9.999999999999980460 ) ;
#13168=ORIENTED_EDGE ( 'NONE', *, *, #685, .F. ) ;
#13197=UNCERTAINTY_MEASURE_WITH_UNIT (LENGTH_MEASURE( 1.000000000000000082E-05 ), #9062, 'distance_accuracy_value', 'NONE');
#13208=EDGE_CURVE ( 'NONE', #1881, #2741, #954, .T. ) ;
#13221=CARTESIAN_POINT ( 'NONE',  ( 242.4999999999999716, -80.00000000000007105, 50.00000000000001421 ) ) ;
#13223=CARTESIAN_POINT ( 'NONE',  ( 222.4999999999999147, -85.00000000000009948, 0.000000000000000000 ) ) ;
#13227=CARTESIAN_POINT ( 'NONE',  ( 203.5000000000000000, -85.00000000000007105, 55.00000000000001421 ) ) ;
#13235=CIRCLE ( 'NONE', #3044, 2.500000000000002220 ) ;
#13286=VERTEX_POINT ( 'NONE', #10111 ) ;
#13312=AXIS2_PLACEMENT_3D ( 'NONE', #7486, #859, #3363 ) ;
#13344=VERTEX_POINT ( 'NONE', #11211 ) ;
#13347=EDGE_LOOP ( 'NONE', ( #12080, #7477, #4298, #3223 ) ) ;
#13357=CARTESIAN_POINT ( 'NONE',  ( 197.5000000000000000, -90.00000000000007105, 55.00000000000001421 ) ) ;
#13407=LINE ( 'NONE', #5722, #5264 ) ;
#13411=VERTEX_POINT ( 'NONE', #4825 ) ;
#13412=MANIFOLD_SOLID_BREP ( 'M5 Machine Threads Stud1', #2200 ) ;
#13414=CARTESIAN_POINT ( 'NONE',  ( 242.5000000000000000, -90.00000000000007105, 50.00000000000001421 ) ) ;
#13415=EDGE_LOOP ( 'NONE', ( #6835, #7533, #3632, #11908 ) ) ;
#13432=ORIENTED_EDGE ( 'NONE', *, *, #5877, .F. ) ;
#13450=AXIS2_PLACEMENT_3D ( 'NONE', #13949, #14232, #4164 ) ;
#13468=AXIS2_PLACEMENT_3D ( 'NONE', #11774, #10691, #6182 ) ;
#13500=CARTESIAN_POINT ( 'NONE',  ( 214.9999999999999716, -85.00000000000007105, 0.000000000000000000 ) ) ;
#13507=ORIENTED_EDGE ( 'NONE', *, *, #14193, .T. ) ;
#13542=AXIS2_PLACEMENT_3D ( 'NONE', #6464, #7681, #4289 ) ;
#13560=EDGE_CURVE ( 'NONE', #4926, #6823, #14093, .T. ) ;
#13587=AXIS2_PLACEMENT_3D ( 'NONE', #5669, #127, #1453 ) ;
#13629=CARTESIAN_POINT ( 'NONE',  ( 229.9999999999999432, -85.00000000000007105, 170.0000000000000000 ) ) ;
#13660=VECTOR ( 'NONE', #11800, 1000.000000000000000 ) ;
#13676=DIRECTION ( 'NONE',  ( 0.000000000000000000, 0.000000000000000000, 1.000000000000000000 ) ) ;
#13684=DIRECTION ( 'NONE',  ( -1.000000000000000000, 0.000000000000000000, -0.000000000000000000 ) ) ;
#13689=DIRECTION ( 'NONE',  ( -0.000000000000000000, -0.000000000000000000, 1.000000000000000000 ) ) ;
#13698=DIRECTION ( 'NONE',  ( 1.000000000000000000, 0.000000000000000000, 0.000000000000000000 ) ) ;
#13771=ORIENTED_EDGE ( 'NONE', *, *, #8605, .T. ) ;
#13782=CARTESIAN_POINT ( 'NONE',  ( 211.3397459621556038, -90.00000000000007105, 170.0000000000000000 ) ) ;
#13791=FACE_BOUND ( 'NONE', #2310, .T. ) ;
#13792=ADVANCED_FACE ( 'NONE', ( #3230 ), #11256, .T. ) ;
#13824=DIRECTION ( 'NONE',  ( -1.000000000000000000, 0.000000000000000000, -0.000000000000000000 ) ) ;
#13827=ORIENTED_EDGE ( 'NONE', *, *, #685, .T. ) ;
#13881=VERTEX_POINT ( 'NONE', #2693 ) ;
#13896=CARTESIAN_POINT ( 'NONE',  ( 233.8499999999999375, -85.00000000000007105, 55.00000000000001421 ) ) ;
#13911=ORIENTED_EDGE ( 'NONE', *, *, #7170, .F. ) ;
#13949=CARTESIAN_POINT ( 'NONE',  ( 219.9999999999999147, -85.00000000000009948, -18.00000000000000355 ) ) ;
#13969=DIRECTION ( 'NONE',  ( -0.000000000000000000, 0.000000000000000000, 1.000000000000000000 ) ) ;
#13993=DIRECTION ( 'NONE',  ( 0.000000000000000000, 0.000000000000000000, 1.000000000000000000 ) ) ;
#13997=EDGE_CURVE ( 'NONE', #682, #11608, #9076, .T. ) ;
#14014=AXIS2_PLACEMENT_3D ( 'NONE', #8403, #12613, #3775 ) ;
#14036=DIRECTION ( 'NONE',  ( -1.000000000000000000, 0.000000000000000000, 0.000000000000000000 ) ) ;
#14039=AXIS2_PLACEMENT_3D ( 'NONE', #10508, #9418, #5077 ) ;
#14082=AXIS2_PLACEMENT_3D ( 'NONE', #540, #13689, #12540 ) ;
#14093=LINE ( 'NONE', #12857, #5072 ) ;
#14096=CARTESIAN_POINT ( 'NONE',  ( 203.5000000000000000, -85.00000000000007105, 55.00000000000001421 ) ) ;
#14098=ORIENTED_EDGE ( 'NONE', *, *, #5467, .T. ) ;
#14099=DIRECTION ( 'NONE',  ( -0.000000000000000000, 0.000000000000000000, 1.000000000000000000 ) ) ;
#14140=CARTESIAN_POINT ( 'NONE',  ( 197.5000000000000000, -90.00000000000007105, 50.00000000000001421 ) ) ;
#14159=CARTESIAN_POINT ( 'NONE',  ( 200.8500000000000227, -85.00000000000007105, 55.00000000000001421 ) ) ;
#14185=FACE_BOUND ( 'NONE', #10687, .T. ) ;
#14193=EDGE_CURVE ( 'NONE', #2276, #3217, #10332, .T. ) ;
#14211=DIRECTION ( 'NONE',  ( 0.000000000000000000, 0.000000000000000000, 1.000000000000000000 ) ) ;
#14232=DIRECTION ( 'NONE',  ( -0.000000000000000000, -0.000000000000000000, 1.000000000000000000 ) ) ;
#14418=COLOUR_RGB('Off White',0.89,0.88,0.83);
#14419=FILL_AREA_STYLE_COLOUR('',#14418);
#14420=FILL_AREA_STYLE('',(#14419));
#14421=SURFACE_STYLE_FILL_AREA(#14420);
#14422=SURFACE_SIDE_STYLE('',(#14421));
#14423=SURFACE_STYLE_USAGE(.BOTH.,#14422);
#14424=PRESENTATION_STYLE_ASSIGNMENT((#14423));
ENDSEC;
END-ISO-10303-21;
